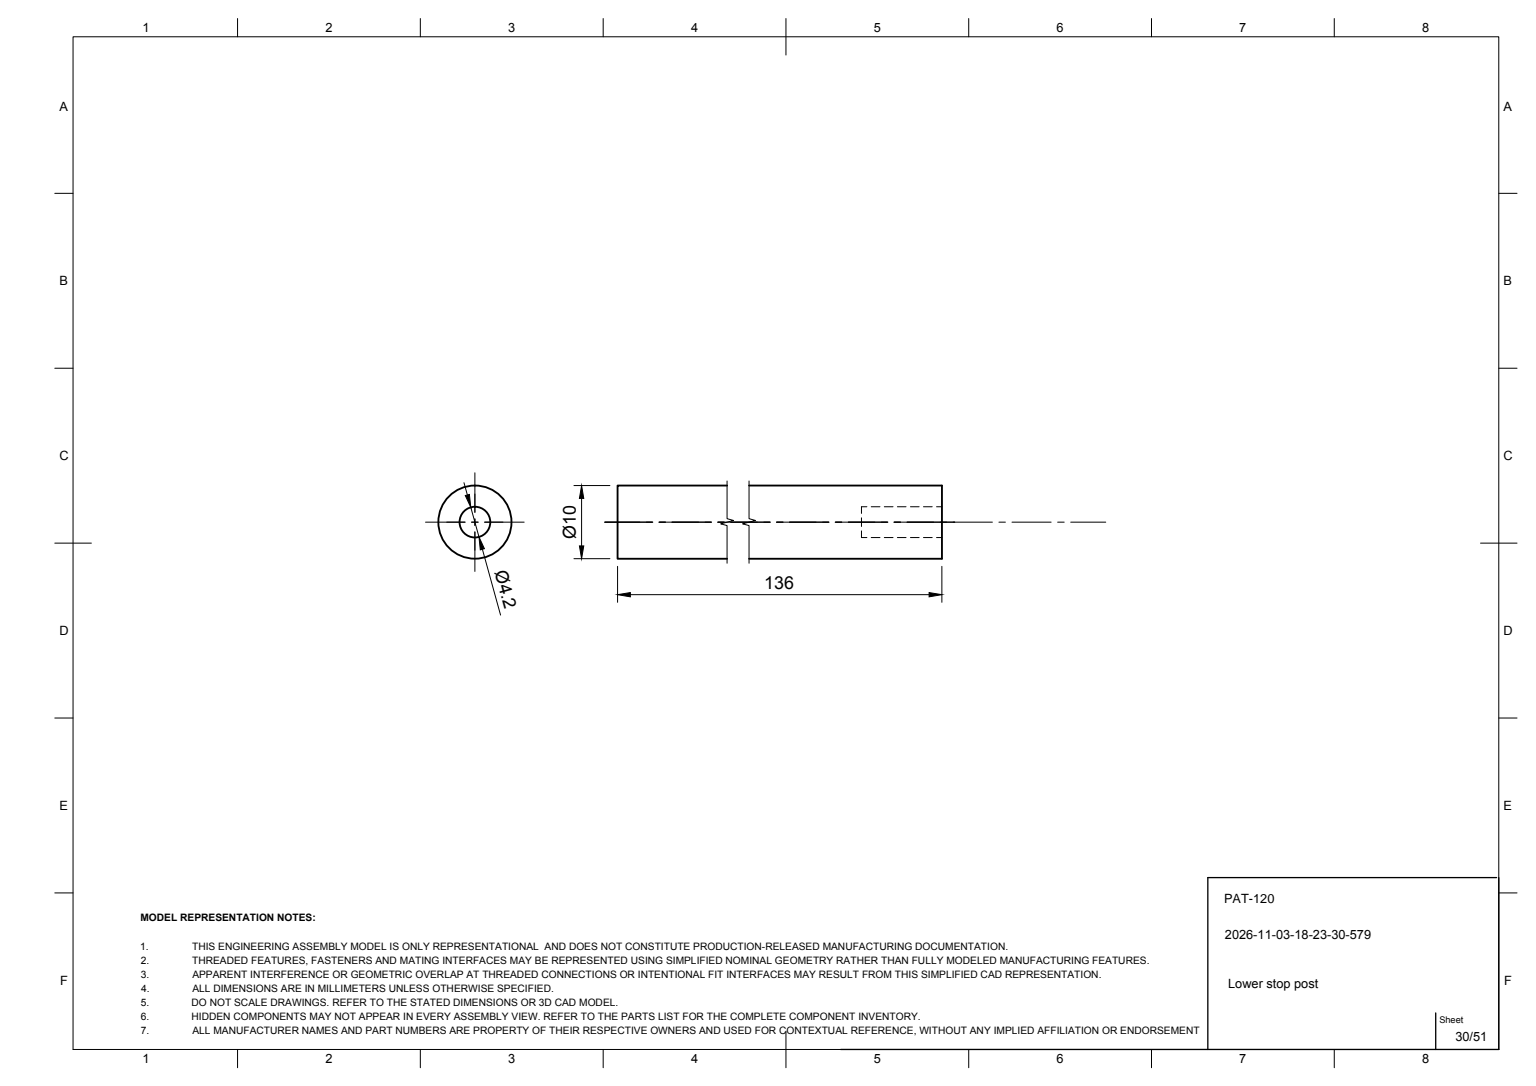
ISO-10303-21;
HEADER;
/* Generated by software containing ST-Developer
 * from STEP Tools, Inc. (www.steptools.com) 
 */

FILE_DESCRIPTION(
/* description */ ('Vibration shaker table dummy'),
/* implementation_level */ '2;1');

FILE_NAME(
/* name */ 'Lower stop post.step',
/* time_stamp */ '2026-10-27T10:55:14-07:00',
/* author */ (''),
/* organization */ (''),
/* preprocessor_version */ 'ST-DEVELOPER v20.2',
/* originating_system */ 'Autodesk Translation Framework v15.17.0.0',
/* authorisation */ '');

FILE_SCHEMA (('AUTOMOTIVE_DESIGN { 1 0 10303 214 3 1 1 }'));
ENDSEC;

DATA;
#10=MECHANICAL_DESIGN_GEOMETRIC_PRESENTATION_REPRESENTATION('',(#711),#22394);
#619=SHAPE_REPRESENTATION_RELATIONSHIP('SRR','None',#22665,#665);
#665=ADVANCED_BREP_SHAPE_REPRESENTATION('',(#757),#22371);
#711=STYLED_ITEM('',(#22947),#757);
#757=MANIFOLD_SOLID_BREP('Body1',#9229);
#943=FACE_BOUND('',#2272,.T.);
#1212=PLANE('',#10279);
#1213=PLANE('',#10283);
#1214=PLANE('',#10284);
#1601=FACE_OUTER_BOUND('',#2267,.T.);
#1602=FACE_OUTER_BOUND('',#2268,.T.);
#1603=FACE_OUTER_BOUND('',#2269,.T.);
#1604=FACE_OUTER_BOUND('',#2270,.T.);
#1605=FACE_OUTER_BOUND('',#2271,.T.);
#2267=EDGE_LOOP('',(#7422,#7423,#7424,#7425));
#2268=EDGE_LOOP('',(#7426));
#2269=EDGE_LOOP('',(#7427,#7428,#7429,#7430));
#2270=EDGE_LOOP('',(#7431));
#2271=EDGE_LOOP('',(#7432));
#2272=EDGE_LOOP('',(#7433));
#2974=LINE('',#20999,#3593);
#2975=LINE('',#21006,#3594);
#3593=VECTOR('',#12338,0.21);
#3594=VECTOR('',#12347,0.5);
#4092=CIRCLE('',#10277,0.21);
#4093=CIRCLE('',#10278,0.21);
#4094=CIRCLE('',#10281,0.5);
#4095=CIRCLE('',#10282,0.5);
#4759=VERTEX_POINT('',#20996);
#4760=VERTEX_POINT('',#20998);
#4761=VERTEX_POINT('',#21003);
#4762=VERTEX_POINT('',#21005);
#5704=EDGE_CURVE('',#4759,#4759,#4092,.T.);
#5705=EDGE_CURVE('',#4759,#4760,#2974,.T.);
#5706=EDGE_CURVE('',#4760,#4760,#4093,.T.);
#5707=EDGE_CURVE('',#4761,#4761,#4094,.T.);
#5708=EDGE_CURVE('',#4761,#4762,#2975,.T.);
#5709=EDGE_CURVE('',#4762,#4762,#4095,.T.);
#7422=ORIENTED_EDGE('',*,*,#5704,.F.);
#7423=ORIENTED_EDGE('',*,*,#5705,.T.);
#7424=ORIENTED_EDGE('',*,*,#5706,.T.);
#7425=ORIENTED_EDGE('',*,*,#5705,.F.);
#7426=ORIENTED_EDGE('',*,*,#5706,.F.);
#7427=ORIENTED_EDGE('',*,*,#5707,.F.);
#7428=ORIENTED_EDGE('',*,*,#5708,.T.);
#7429=ORIENTED_EDGE('',*,*,#5709,.T.);
#7430=ORIENTED_EDGE('',*,*,#5708,.F.);
#7431=ORIENTED_EDGE('',*,*,#5707,.T.);
#7432=ORIENTED_EDGE('',*,*,#5709,.F.);
#7433=ORIENTED_EDGE('',*,*,#5704,.T.);
#8610=CYLINDRICAL_SURFACE('',#10276,0.21);
#8611=CYLINDRICAL_SURFACE('',#10280,0.5);
#8966=ADVANCED_FACE('',(#1601),#8610,.F.);
#8967=ADVANCED_FACE('',(#1602),#1212,.F.);
#8968=ADVANCED_FACE('',(#1603),#8611,.T.);
#8969=ADVANCED_FACE('',(#1604),#1213,.T.);
#8970=ADVANCED_FACE('',(#1605,#943),#1214,.F.);
#9229=CLOSED_SHELL('',(#8966,#8967,#8968,#8969,#8970));
#10275=AXIS2_PLACEMENT_3D('',#20994,#12332,#12333);
#10276=AXIS2_PLACEMENT_3D('',#20995,#12334,#12335);
#10277=AXIS2_PLACEMENT_3D('',#20997,#12336,#12337);
#10278=AXIS2_PLACEMENT_3D('',#21000,#12339,#12340);
#10279=AXIS2_PLACEMENT_3D('',#21001,#12341,#12342);
#10280=AXIS2_PLACEMENT_3D('',#21002,#12343,#12344);
#10281=AXIS2_PLACEMENT_3D('',#21004,#12345,#12346);
#10282=AXIS2_PLACEMENT_3D('',#21007,#12348,#12349);
#10283=AXIS2_PLACEMENT_3D('',#21008,#12350,#12351);
#10284=AXIS2_PLACEMENT_3D('',#21009,#12352,#12353);
#12332=DIRECTION('axis',(0.,0.,1.));
#12333=DIRECTION('refdir',(1.,0.,0.));
#12334=DIRECTION('center_axis',(0.,0.,1.));
#12335=DIRECTION('ref_axis',(1.,0.,0.));
#12336=DIRECTION('center_axis',(0.,0.,1.));
#12337=DIRECTION('ref_axis',(1.,0.,0.));
#12338=DIRECTION('',(0.,0.,1.));
#12339=DIRECTION('center_axis',(0.,0.,1.));
#12340=DIRECTION('ref_axis',(1.,0.,0.));
#12341=DIRECTION('center_axis',(0.,0.,1.));
#12342=DIRECTION('ref_axis',(1.,0.,0.));
#12343=DIRECTION('center_axis',(0.,0.,1.));
#12344=DIRECTION('ref_axis',(1.,0.,0.));
#12345=DIRECTION('center_axis',(0.,0.,1.));
#12346=DIRECTION('ref_axis',(1.,0.,0.));
#12347=DIRECTION('',(0.,0.,-1.));
#12348=DIRECTION('center_axis',(0.,0.,1.));
#12349=DIRECTION('ref_axis',(1.,0.,0.));
#12350=DIRECTION('center_axis',(0.,0.,1.));
#12351=DIRECTION('ref_axis',(1.,0.,0.));
#12352=DIRECTION('center_axis',(0.,0.,1.));
#12353=DIRECTION('ref_axis',(1.,0.,0.));
#20994=CARTESIAN_POINT('',(0.,0.,0.));
#20995=CARTESIAN_POINT('Origin',(0.,-6.,-0.1));
#20996=CARTESIAN_POINT('',(-0.21,-6.,0.));
#20997=CARTESIAN_POINT('Origin',(0.,-6.,0.));
#20998=CARTESIAN_POINT('',(-0.21,-6.,1.1));
#20999=CARTESIAN_POINT('',(-0.21,-6.,-0.1));
#21000=CARTESIAN_POINT('Origin',(0.,-6.,1.1));
#21001=CARTESIAN_POINT('Origin',(0.,-6.,1.1));
#21002=CARTESIAN_POINT('Origin',(0.,-6.,0.));
#21003=CARTESIAN_POINT('',(-0.5,-6.,13.6));
#21004=CARTESIAN_POINT('Origin',(0.,-6.,13.6));
#21005=CARTESIAN_POINT('',(-0.5,-6.,0.));
#21006=CARTESIAN_POINT('',(-0.5,-6.,0.));
#21007=CARTESIAN_POINT('Origin',(0.,-6.,0.));
#21008=CARTESIAN_POINT('Origin',(0.,-6.,13.6));
#21009=CARTESIAN_POINT('Origin',(0.,-6.,0.));
#22320=UNCERTAINTY_MEASURE_WITH_UNIT(LENGTH_MEASURE(0.001),#22395,
'DISTANCE_ACCURACY_VALUE',
'Maximum model space distance between geometric entities at asserted c
onnectivities');
#22343=UNCERTAINTY_MEASURE_WITH_UNIT(LENGTH_MEASURE(0.001),#22395,
'DISTANCE_ACCURACY_VALUE',
'Maximum model space distance between geometric entities at asserted c
onnectivities');
#22371=(
GEOMETRIC_REPRESENTATION_CONTEXT(3)
GLOBAL_UNCERTAINTY_ASSIGNED_CONTEXT((#22320))
GLOBAL_UNIT_ASSIGNED_CONTEXT((#22395,#22397,#22398))
REPRESENTATION_CONTEXT('','3D')
);
#22394=(
GEOMETRIC_REPRESENTATION_CONTEXT(3)
GLOBAL_UNCERTAINTY_ASSIGNED_CONTEXT((#22343))
GLOBAL_UNIT_ASSIGNED_CONTEXT((#22395,#22397,#22398))
REPRESENTATION_CONTEXT('','3D')
);
#22395=(
LENGTH_UNIT()
NAMED_UNIT(*)
SI_UNIT(.CENTI.,.METRE.)
);
#22397=(
NAMED_UNIT(*)
PLANE_ANGLE_UNIT()
SI_UNIT($,.RADIAN.)
);
#22398=(
NAMED_UNIT(*)
SI_UNIT($,.STERADIAN.)
SOLID_ANGLE_UNIT()
);
#22426=SHAPE_DEFINITION_REPRESENTATION(#22476,#22665);
#22476=PRODUCT_DEFINITION_SHAPE('',$,#22716);
#22665=SHAPE_REPRESENTATION('',(#10275),#22371);
#22688=PRODUCT_DEFINITION_CONTEXT('part definition',#22840,'design');
#22716=PRODUCT_DEFINITION('Lower stop post','Lower stop post',#22766,#22688);
#22766=PRODUCT_DEFINITION_FORMATION('',$,#22869);
#22840=APPLICATION_CONTEXT(
'Core Data for Automotive Mechanical Design Process');
#22841=PRODUCT_CONTEXT('part definition',#22840,'mechanical');
#22869=PRODUCT('Lower stop post','Lower stop post','Lower stop post',(#22841));
#22941=COLOUR_RGB('Light Blue',0.38,0.62,0.78);
#22942=FILL_AREA_STYLE_COLOUR('',#22941);
#22943=FILL_AREA_STYLE('',(#22942));
#22944=SURFACE_STYLE_FILL_AREA(#22943);
#22945=SURFACE_SIDE_STYLE('',(#22944));
#22946=SURFACE_STYLE_USAGE(.BOTH.,#22945);
#22947=PRESENTATION_STYLE_ASSIGNMENT((#22946));
ENDSEC;
END-ISO-10303-21;
